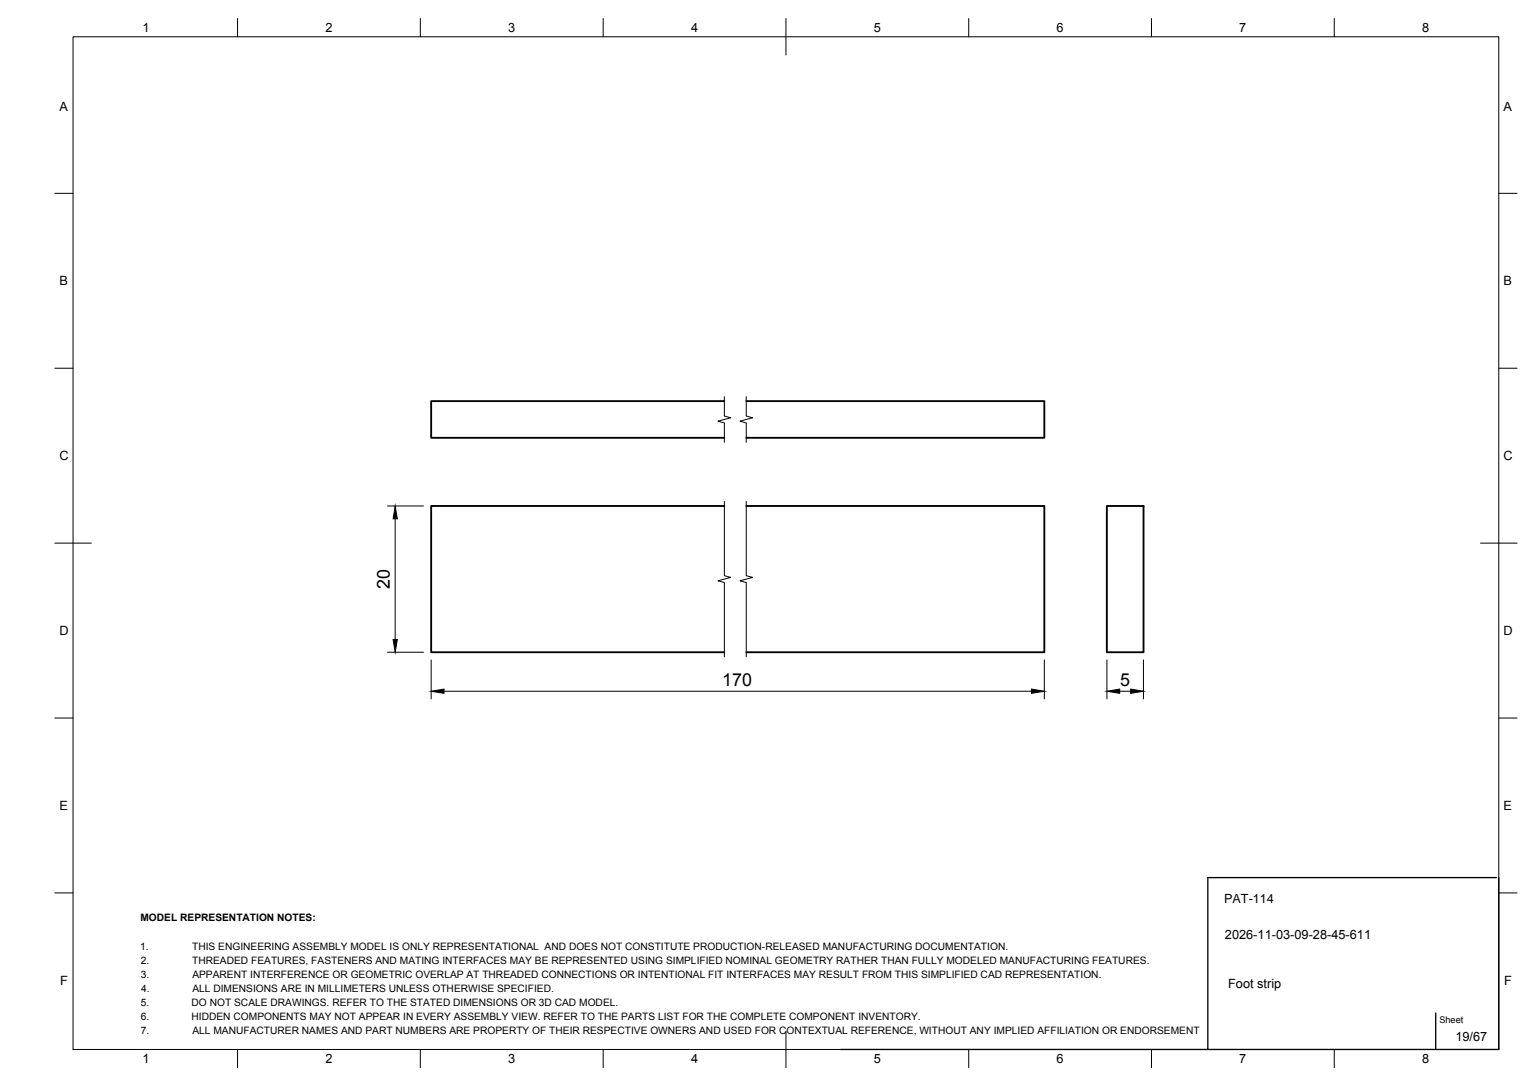
ISO-10303-21;
HEADER;
/* Generated by software containing ST-Developer
 * from STEP Tools, Inc. (www.steptools.com) 
 */

FILE_DESCRIPTION(
/* description */ ('Two-stage gear reducer in split housing'),
/* implementation_level */ '2;1');

FILE_NAME(
/* name */ 'Foot strip.step',
/* time_stamp */ '2026-10-28T03:22:31-07:00',
/* author */ (''),
/* organization */ (''),
/* preprocessor_version */ 'ST-DEVELOPER v20.2',
/* originating_system */ 'Autodesk Translation Framework v15.17.0.0',
/* authorisation */ '');

FILE_SCHEMA (('AUTOMOTIVE_DESIGN { 1 0 10303 214 3 1 1 }'));
ENDSEC;

DATA;
#10=MECHANICAL_DESIGN_GEOMETRIC_PRESENTATION_REPRESENTATION('',(#1248),#73366);
#1136=SHAPE_REPRESENTATION_RELATIONSHIP('SRR','None',#73623,#1192);
#1192=ADVANCED_BREP_SHAPE_REPRESENTATION('',(#1319),#73319);
#1248=STYLED_ITEM('',(#73974),#1319);
#1319=MANIFOLD_SOLID_BREP('Body1',#16136);
#1732=PLANE('',#17379);
#1733=PLANE('',#17380);
#1734=PLANE('',#17381);
#1735=PLANE('',#17382);
#1736=PLANE('',#17383);
#1737=PLANE('',#17384);
#2272=FACE_OUTER_BOUND('',#3329,.T.);
#2273=FACE_OUTER_BOUND('',#3330,.T.);
#2274=FACE_OUTER_BOUND('',#3331,.T.);
#2275=FACE_OUTER_BOUND('',#3332,.T.);
#2276=FACE_OUTER_BOUND('',#3333,.T.);
#2277=FACE_OUTER_BOUND('',#3334,.T.);
#3329=EDGE_LOOP('',(#11707,#11708,#11709,#11710));
#3330=EDGE_LOOP('',(#11711,#11712,#11713,#11714));
#3331=EDGE_LOOP('',(#11715,#11716,#11717,#11718));
#3332=EDGE_LOOP('',(#11719,#11720,#11721,#11722));
#3333=EDGE_LOOP('',(#11723,#11724,#11725,#11726));
#3334=EDGE_LOOP('',(#11727,#11728,#11729,#11730));
#4376=LINE('',#24064,#5400);
#4377=LINE('',#24066,#5401);
#4378=LINE('',#24068,#5402);
#4379=LINE('',#24069,#5403);
#4380=LINE('',#24072,#5404);
#4381=LINE('',#24074,#5405);
#4382=LINE('',#24075,#5406);
#4383=LINE('',#24078,#5407);
#4384=LINE('',#24080,#5408);
#4385=LINE('',#24081,#5409);
#4386=LINE('',#24083,#5410);
#4387=LINE('',#24084,#5411);
#5400=VECTOR('',#19914,1.);
#5401=VECTOR('',#19915,1.);
#5402=VECTOR('',#19916,1.);
#5403=VECTOR('',#19917,1.);
#5404=VECTOR('',#19920,1.);
#5405=VECTOR('',#19921,1.);
#5406=VECTOR('',#19922,1.);
#5407=VECTOR('',#19925,1.);
#5408=VECTOR('',#19926,1.);
#5409=VECTOR('',#19927,1.);
#5410=VECTOR('',#19930,1.);
#5411=VECTOR('',#19931,1.);
#7224=VERTEX_POINT('',#24062);
#7225=VERTEX_POINT('',#24063);
#7226=VERTEX_POINT('',#24065);
#7227=VERTEX_POINT('',#24067);
#7228=VERTEX_POINT('',#24071);
#7229=VERTEX_POINT('',#24073);
#7230=VERTEX_POINT('',#24077);
#7231=VERTEX_POINT('',#24079);
#8907=EDGE_CURVE('',#7224,#7225,#4376,.T.);
#8908=EDGE_CURVE('',#7225,#7226,#4377,.T.);
#8909=EDGE_CURVE('',#7227,#7226,#4378,.T.);
#8910=EDGE_CURVE('',#7224,#7227,#4379,.T.);
#8911=EDGE_CURVE('',#7228,#7224,#4380,.T.);
#8912=EDGE_CURVE('',#7229,#7227,#4381,.T.);
#8913=EDGE_CURVE('',#7228,#7229,#4382,.T.);
#8914=EDGE_CURVE('',#7230,#7228,#4383,.T.);
#8915=EDGE_CURVE('',#7231,#7229,#4384,.T.);
#8916=EDGE_CURVE('',#7230,#7231,#4385,.T.);
#8917=EDGE_CURVE('',#7225,#7230,#4386,.T.);
#8918=EDGE_CURVE('',#7226,#7231,#4387,.T.);
#11707=ORIENTED_EDGE('',*,*,#8907,.T.);
#11708=ORIENTED_EDGE('',*,*,#8908,.T.);
#11709=ORIENTED_EDGE('',*,*,#8909,.F.);
#11710=ORIENTED_EDGE('',*,*,#8910,.F.);
#11711=ORIENTED_EDGE('',*,*,#8911,.T.);
#11712=ORIENTED_EDGE('',*,*,#8910,.T.);
#11713=ORIENTED_EDGE('',*,*,#8912,.F.);
#11714=ORIENTED_EDGE('',*,*,#8913,.F.);
#11715=ORIENTED_EDGE('',*,*,#8914,.T.);
#11716=ORIENTED_EDGE('',*,*,#8913,.T.);
#11717=ORIENTED_EDGE('',*,*,#8915,.F.);
#11718=ORIENTED_EDGE('',*,*,#8916,.F.);
#11719=ORIENTED_EDGE('',*,*,#8917,.T.);
#11720=ORIENTED_EDGE('',*,*,#8916,.T.);
#11721=ORIENTED_EDGE('',*,*,#8918,.F.);
#11722=ORIENTED_EDGE('',*,*,#8908,.F.);
#11723=ORIENTED_EDGE('',*,*,#8918,.T.);
#11724=ORIENTED_EDGE('',*,*,#8915,.T.);
#11725=ORIENTED_EDGE('',*,*,#8912,.T.);
#11726=ORIENTED_EDGE('',*,*,#8909,.T.);
#11727=ORIENTED_EDGE('',*,*,#8917,.F.);
#11728=ORIENTED_EDGE('',*,*,#8907,.F.);
#11729=ORIENTED_EDGE('',*,*,#8911,.F.);
#11730=ORIENTED_EDGE('',*,*,#8914,.F.);
#15479=ADVANCED_FACE('',(#2272),#1732,.T.);
#15480=ADVANCED_FACE('',(#2273),#1733,.T.);
#15481=ADVANCED_FACE('',(#2274),#1734,.T.);
#15482=ADVANCED_FACE('',(#2275),#1735,.T.);
#15483=ADVANCED_FACE('',(#2276),#1736,.T.);
#15484=ADVANCED_FACE('',(#2277),#1737,.F.);
#16136=CLOSED_SHELL('',(#15479,#15480,#15481,#15482,#15483,#15484));
#17378=AXIS2_PLACEMENT_3D('',#24060,#19910,#19911);
#17379=AXIS2_PLACEMENT_3D('',#24061,#19912,#19913);
#17380=AXIS2_PLACEMENT_3D('',#24070,#19918,#19919);
#17381=AXIS2_PLACEMENT_3D('',#24076,#19923,#19924);
#17382=AXIS2_PLACEMENT_3D('',#24082,#19928,#19929);
#17383=AXIS2_PLACEMENT_3D('',#24085,#19932,#19933);
#17384=AXIS2_PLACEMENT_3D('',#24086,#19934,#19935);
#19910=DIRECTION('axis',(0.,0.,1.));
#19911=DIRECTION('refdir',(1.,0.,0.));
#19912=DIRECTION('center_axis',(0.,1.,0.));
#19913=DIRECTION('ref_axis',(-1.,0.,0.));
#19914=DIRECTION('',(-1.,0.,0.));
#19915=DIRECTION('',(0.,0.,1.));
#19916=DIRECTION('',(-1.,0.,0.));
#19917=DIRECTION('',(0.,0.,1.));
#19918=DIRECTION('center_axis',(1.,0.,0.));
#19919=DIRECTION('ref_axis',(0.,1.,0.));
#19920=DIRECTION('',(0.,1.,0.));
#19921=DIRECTION('',(0.,1.,0.));
#19922=DIRECTION('',(0.,0.,1.));
#19923=DIRECTION('center_axis',(0.,-1.,0.));
#19924=DIRECTION('ref_axis',(1.,0.,0.));
#19925=DIRECTION('',(1.,0.,0.));
#19926=DIRECTION('',(1.,0.,0.));
#19927=DIRECTION('',(0.,0.,1.));
#19928=DIRECTION('center_axis',(-1.,0.,0.));
#19929=DIRECTION('ref_axis',(0.,-1.,0.));
#19930=DIRECTION('',(0.,-1.,0.));
#19931=DIRECTION('',(0.,-1.,0.));
#19932=DIRECTION('center_axis',(0.,0.,1.));
#19933=DIRECTION('ref_axis',(1.,0.,0.));
#19934=DIRECTION('center_axis',(0.,0.,1.));
#19935=DIRECTION('ref_axis',(1.,0.,0.));
#24060=CARTESIAN_POINT('',(0.,0.,0.));
#24061=CARTESIAN_POINT('Origin',(-3.5,8.5,-0.5));
#24062=CARTESIAN_POINT('',(-3.5,8.5,-0.5));
#24063=CARTESIAN_POINT('',(-5.5,8.5,-0.5));
#24064=CARTESIAN_POINT('',(-3.5,8.5,-0.5));
#24065=CARTESIAN_POINT('',(-5.5,8.5,0.));
#24066=CARTESIAN_POINT('',(-5.5,8.5,-0.5));
#24067=CARTESIAN_POINT('',(-3.5,8.5,0.));
#24068=CARTESIAN_POINT('',(-3.5,8.5,0.));
#24069=CARTESIAN_POINT('',(-3.5,8.5,-0.5));
#24070=CARTESIAN_POINT('Origin',(-3.5,-8.5,-0.5));
#24071=CARTESIAN_POINT('',(-3.5,-8.5,-0.5));
#24072=CARTESIAN_POINT('',(-3.5,-8.5,-0.5));
#24073=CARTESIAN_POINT('',(-3.5,-8.5,0.));
#24074=CARTESIAN_POINT('',(-3.5,-8.5,0.));
#24075=CARTESIAN_POINT('',(-3.5,-8.5,-0.5));
#24076=CARTESIAN_POINT('Origin',(-5.5,-8.5,-0.5));
#24077=CARTESIAN_POINT('',(-5.5,-8.5,-0.5));
#24078=CARTESIAN_POINT('',(-5.5,-8.5,-0.5));
#24079=CARTESIAN_POINT('',(-5.5,-8.5,0.));
#24080=CARTESIAN_POINT('',(-5.5,-8.5,0.));
#24081=CARTESIAN_POINT('',(-5.5,-8.5,-0.5));
#24082=CARTESIAN_POINT('Origin',(-5.5,8.5,-0.5));
#24083=CARTESIAN_POINT('',(-5.5,8.5,-0.5));
#24084=CARTESIAN_POINT('',(-5.5,8.5,0.));
#24085=CARTESIAN_POINT('Origin',(-4.5,0.,0.));
#24086=CARTESIAN_POINT('Origin',(-4.5,0.,-0.5));
#73255=UNCERTAINTY_MEASURE_WITH_UNIT(LENGTH_MEASURE(0.001),#73367,
'DISTANCE_ACCURACY_VALUE',
'Maximum model space distance between geometric entities at asserted c
onnectivities');
#73302=UNCERTAINTY_MEASURE_WITH_UNIT(LENGTH_MEASURE(0.001),#73367,
'DISTANCE_ACCURACY_VALUE',
'Maximum model space distance between geometric entities at asserted c
onnectivities');
#73319=(
GEOMETRIC_REPRESENTATION_CONTEXT(3)
GLOBAL_UNCERTAINTY_ASSIGNED_CONTEXT((#73255))
GLOBAL_UNIT_ASSIGNED_CONTEXT((#73367,#73369,#73370))
REPRESENTATION_CONTEXT('','3D')
);
#73366=(
GEOMETRIC_REPRESENTATION_CONTEXT(3)
GLOBAL_UNCERTAINTY_ASSIGNED_CONTEXT((#73302))
GLOBAL_UNIT_ASSIGNED_CONTEXT((#73367,#73369,#73370))
REPRESENTATION_CONTEXT('','3D')
);
#73367=(
LENGTH_UNIT()
NAMED_UNIT(*)
SI_UNIT(.CENTI.,.METRE.)
);
#73369=(
NAMED_UNIT(*)
PLANE_ANGLE_UNIT()
SI_UNIT($,.RADIAN.)
);
#73370=(
NAMED_UNIT(*)
SI_UNIT($,.STERADIAN.)
SOLID_ANGLE_UNIT()
);
#73387=SHAPE_DEFINITION_REPRESENTATION(#73450,#73623);
#73450=PRODUCT_DEFINITION_SHAPE('',$,#73687);
#73623=SHAPE_REPRESENTATION('',(#17378),#73319);
#73670=PRODUCT_DEFINITION_CONTEXT('part definition',#73861,'design');
#73687=PRODUCT_DEFINITION('Foot strip','Foot strip',#73750,#73670);
#73750=PRODUCT_DEFINITION_FORMATION('',$,#73879);
#73861=APPLICATION_CONTEXT(
'Core Data for Automotive Mechanical Design Process');
#73862=PRODUCT_CONTEXT('part definition',#73861,'mechanical');
#73879=PRODUCT('Foot strip','Foot strip','Foot strip',(#73862));
#73968=COLOUR_RGB('Light Blue',0.38,0.62,0.78);
#73969=FILL_AREA_STYLE_COLOUR('',#73968);
#73970=FILL_AREA_STYLE('',(#73969));
#73971=SURFACE_STYLE_FILL_AREA(#73970);
#73972=SURFACE_SIDE_STYLE('',(#73971));
#73973=SURFACE_STYLE_USAGE(.BOTH.,#73972);
#73974=PRESENTATION_STYLE_ASSIGNMENT((#73973));
ENDSEC;
END-ISO-10303-21;
